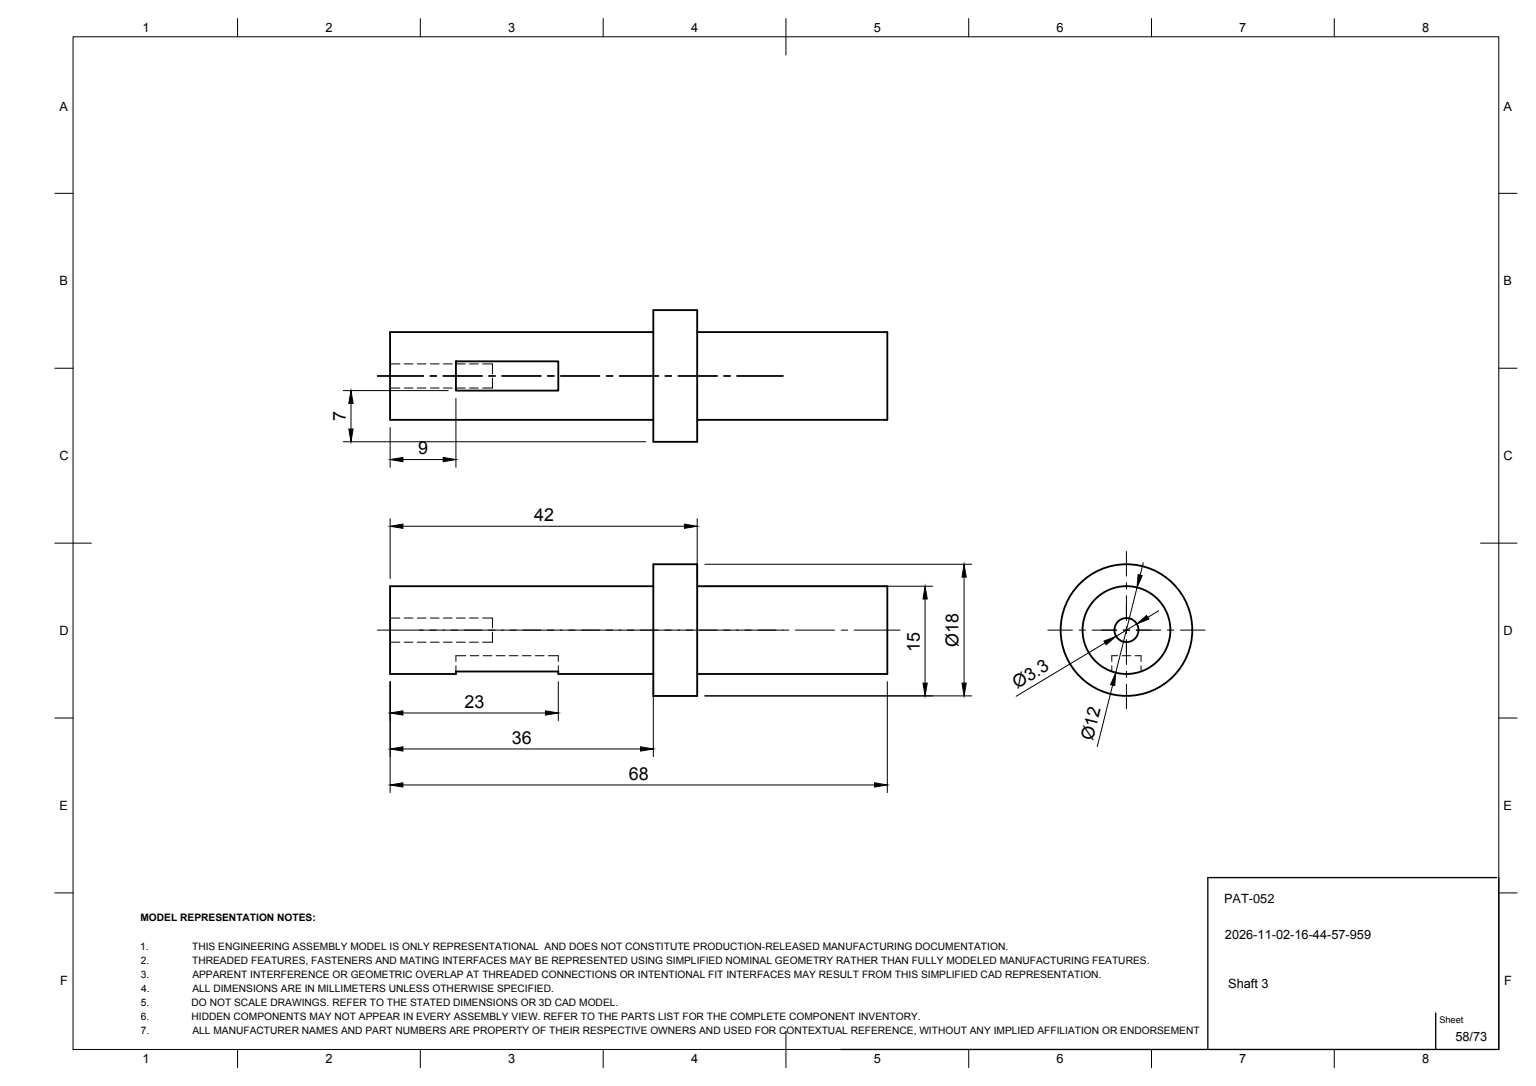
ISO-10303-21;
HEADER;
/* Generated by software containing ST-Developer
 * from STEP Tools, Inc. (www.steptools.com) 
 */

FILE_DESCRIPTION(
/* description */ ('Hand-crank gear train demonstrator'),
/* implementation_level */ '2;1');

FILE_NAME(
/* name */ 'Shaft 3.step',
/* time_stamp */ '2026-10-28T03:22:13-07:00',
/* author */ (''),
/* organization */ (''),
/* preprocessor_version */ 'ST-DEVELOPER v20.2',
/* originating_system */ 'Autodesk Translation Framework v15.17.0.0',
/* authorisation */ '');

FILE_SCHEMA (('AUTOMOTIVE_DESIGN { 1 0 10303 214 3 1 1 }'));
ENDSEC;

DATA;
#10=MECHANICAL_DESIGN_GEOMETRIC_PRESENTATION_REPRESENTATION('',(#1248),#62758);
#1105=SHAPE_REPRESENTATION_RELATIONSHIP('SRR','None',#63082,#1169);
#1169=ADVANCED_BREP_SHAPE_REPRESENTATION('',(#1323),#62736);
#1248=STYLED_ITEM('',(#63462),#1323);
#1323=MANIFOLD_SOLID_BREP('Body1',#16432);
#1586=FACE_BOUND('',#3853,.T.);
#1587=FACE_BOUND('',#3855,.T.);
#1588=FACE_BOUND('',#3859,.T.);
#1589=FACE_BOUND('',#3861,.T.);
#1957=PLANE('',#18208);
#1958=PLANE('',#18209);
#1959=PLANE('',#18210);
#1960=PLANE('',#18212);
#1961=PLANE('',#18213);
#1962=PLANE('',#18214);
#1963=PLANE('',#18216);
#1964=PLANE('',#18219);
#1965=PLANE('',#18227);
#1966=PLANE('',#18228);
#2665=FACE_OUTER_BOUND('',#3845,.T.);
#2666=FACE_OUTER_BOUND('',#3846,.T.);
#2667=FACE_OUTER_BOUND('',#3847,.T.);
#2668=FACE_OUTER_BOUND('',#3848,.T.);
#2669=FACE_OUTER_BOUND('',#3849,.T.);
#2670=FACE_OUTER_BOUND('',#3850,.T.);
#2671=FACE_OUTER_BOUND('',#3851,.T.);
#2672=FACE_OUTER_BOUND('',#3852,.T.);
#2673=FACE_OUTER_BOUND('',#3854,.T.);
#2674=FACE_OUTER_BOUND('',#3856,.T.);
#2675=FACE_OUTER_BOUND('',#3857,.T.);
#2676=FACE_OUTER_BOUND('',#3858,.T.);
#2677=FACE_OUTER_BOUND('',#3860,.T.);
#2678=FACE_OUTER_BOUND('',#3862,.T.);
#3845=EDGE_LOOP('',(#13139,#13140,#13141,#13142));
#3846=EDGE_LOOP('',(#13143));
#3847=EDGE_LOOP('',(#13144,#13145,#13146,#13147));
#3848=EDGE_LOOP('',(#13148,#13149,#13150,#13151));
#3849=EDGE_LOOP('',(#13152,#13153,#13154,#13155));
#3850=EDGE_LOOP('',(#13156,#13157,#13158,#13159));
#3851=EDGE_LOOP('',(#13160,#13161,#13162,#13163));
#3852=EDGE_LOOP('',(#13164));
#3853=EDGE_LOOP('',(#13165));
#3854=EDGE_LOOP('',(#13166));
#3855=EDGE_LOOP('',(#13167));
#3856=EDGE_LOOP('',(#13168,#13169,#13170,#13171));
#3857=EDGE_LOOP('',(#13172,#13173,#13174,#13175));
#3858=EDGE_LOOP('',(#13176,#13177,#13178,#13179));
#3859=EDGE_LOOP('',(#13180,#13181,#13182,#13183));
#3860=EDGE_LOOP('',(#13184));
#3861=EDGE_LOOP('',(#13185));
#3862=EDGE_LOOP('',(#13186));
#4955=LINE('',#26595,#6087);
#4956=LINE('',#26601,#6088);
#4957=LINE('',#26603,#6089);
#4958=LINE('',#26605,#6090);
#4959=LINE('',#26606,#6091);
#4960=LINE('',#26611,#6092);
#4961=LINE('',#26612,#6093);
#4962=LINE('',#26615,#6094);
#4963=LINE('',#26617,#6095);
#4964=LINE('',#26618,#6096);
#4965=LINE('',#26620,#6097);
#4966=LINE('',#26634,#6098);
#4967=LINE('',#26637,#6099);
#4968=LINE('',#26642,#6100);
#6087=VECTOR('',#21598,0.164999999999999);
#6088=VECTOR('',#21605,1.);
#6089=VECTOR('',#21606,1.);
#6090=VECTOR('',#21607,1.);
#6091=VECTOR('',#21608,1.);
#6092=VECTOR('',#21613,1.);
#6093=VECTOR('',#21614,1.);
#6094=VECTOR('',#21617,1.);
#6095=VECTOR('',#21618,1.);
#6096=VECTOR('',#21619,1.);
#6097=VECTOR('',#21622,1.);
#6098=VECTOR('',#21641,0.9);
#6099=VECTOR('',#21644,0.6);
#6100=VECTOR('',#21651,0.6);
#6993=CIRCLE('',#18206,0.164999999999999);
#6994=CIRCLE('',#18207,0.164999999999999);
#6995=CIRCLE('',#18211,0.6);
#6996=CIRCLE('',#18215,0.6);
#6997=CIRCLE('',#18217,0.9);
#6998=CIRCLE('',#18218,0.6);
#6999=CIRCLE('',#18220,0.9);
#7000=CIRCLE('',#18221,0.6);
#7001=CIRCLE('',#18224,0.6);
#7002=CIRCLE('',#18226,0.6);
#7994=VERTEX_POINT('',#26592);
#7995=VERTEX_POINT('',#26594);
#7996=VERTEX_POINT('',#26599);
#7997=VERTEX_POINT('',#26600);
#7998=VERTEX_POINT('',#26602);
#7999=VERTEX_POINT('',#26604);
#8000=VERTEX_POINT('',#26608);
#8001=VERTEX_POINT('',#26610);
#8002=VERTEX_POINT('',#26614);
#8003=VERTEX_POINT('',#26616);
#8004=VERTEX_POINT('',#26624);
#8005=VERTEX_POINT('',#26626);
#8006=VERTEX_POINT('',#26629);
#8007=VERTEX_POINT('',#26631);
#8008=VERTEX_POINT('',#26636);
#8009=VERTEX_POINT('',#26640);
#9821=EDGE_CURVE('',#7994,#7994,#6993,.T.);
#9822=EDGE_CURVE('',#7994,#7995,#4955,.T.);
#9823=EDGE_CURVE('',#7995,#7995,#6994,.T.);
#9824=EDGE_CURVE('',#7996,#7997,#4956,.T.);
#9825=EDGE_CURVE('',#7996,#7998,#4957,.T.);
#9826=EDGE_CURVE('',#7999,#7998,#4958,.T.);
#9827=EDGE_CURVE('',#7999,#7997,#4959,.T.);
#9828=EDGE_CURVE('',#7997,#8000,#6995,.T.);
#9829=EDGE_CURVE('',#8001,#7999,#4960,.T.);
#9830=EDGE_CURVE('',#8000,#8001,#4961,.T.);
#9831=EDGE_CURVE('',#8000,#8002,#4962,.T.);
#9832=EDGE_CURVE('',#8001,#8003,#4963,.T.);
#9833=EDGE_CURVE('',#8003,#8002,#4964,.T.);
#9834=EDGE_CURVE('',#7998,#8003,#4965,.T.);
#9835=EDGE_CURVE('',#8002,#7996,#6996,.T.);
#9836=EDGE_CURVE('',#8004,#8004,#6997,.T.);
#9837=EDGE_CURVE('',#8005,#8005,#6998,.T.);
#9838=EDGE_CURVE('',#8006,#8006,#6999,.T.);
#9839=EDGE_CURVE('',#8007,#8007,#7000,.T.);
#9840=EDGE_CURVE('',#8004,#8006,#4966,.T.);
#9841=EDGE_CURVE('',#8007,#8008,#4967,.T.);
#9842=EDGE_CURVE('',#8008,#8008,#7001,.T.);
#9843=EDGE_CURVE('',#8009,#8009,#7002,.T.);
#9844=EDGE_CURVE('',#8009,#8005,#4968,.T.);
#13139=ORIENTED_EDGE('',*,*,#9821,.F.);
#13140=ORIENTED_EDGE('',*,*,#9822,.T.);
#13141=ORIENTED_EDGE('',*,*,#9823,.F.);
#13142=ORIENTED_EDGE('',*,*,#9822,.F.);
#13143=ORIENTED_EDGE('',*,*,#9821,.T.);
#13144=ORIENTED_EDGE('',*,*,#9824,.F.);
#13145=ORIENTED_EDGE('',*,*,#9825,.T.);
#13146=ORIENTED_EDGE('',*,*,#9826,.F.);
#13147=ORIENTED_EDGE('',*,*,#9827,.T.);
#13148=ORIENTED_EDGE('',*,*,#9828,.F.);
#13149=ORIENTED_EDGE('',*,*,#9827,.F.);
#13150=ORIENTED_EDGE('',*,*,#9829,.F.);
#13151=ORIENTED_EDGE('',*,*,#9830,.F.);
#13152=ORIENTED_EDGE('',*,*,#9831,.F.);
#13153=ORIENTED_EDGE('',*,*,#9830,.T.);
#13154=ORIENTED_EDGE('',*,*,#9832,.T.);
#13155=ORIENTED_EDGE('',*,*,#9833,.T.);
#13156=ORIENTED_EDGE('',*,*,#9829,.T.);
#13157=ORIENTED_EDGE('',*,*,#9826,.T.);
#13158=ORIENTED_EDGE('',*,*,#9834,.T.);
#13159=ORIENTED_EDGE('',*,*,#9832,.F.);
#13160=ORIENTED_EDGE('',*,*,#9835,.F.);
#13161=ORIENTED_EDGE('',*,*,#9833,.F.);
#13162=ORIENTED_EDGE('',*,*,#9834,.F.);
#13163=ORIENTED_EDGE('',*,*,#9825,.F.);
#13164=ORIENTED_EDGE('',*,*,#9836,.T.);
#13165=ORIENTED_EDGE('',*,*,#9837,.F.);
#13166=ORIENTED_EDGE('',*,*,#9838,.F.);
#13167=ORIENTED_EDGE('',*,*,#9839,.F.);
#13168=ORIENTED_EDGE('',*,*,#9836,.F.);
#13169=ORIENTED_EDGE('',*,*,#9840,.T.);
#13170=ORIENTED_EDGE('',*,*,#9838,.T.);
#13171=ORIENTED_EDGE('',*,*,#9840,.F.);
#13172=ORIENTED_EDGE('',*,*,#9839,.T.);
#13173=ORIENTED_EDGE('',*,*,#9841,.T.);
#13174=ORIENTED_EDGE('',*,*,#9842,.T.);
#13175=ORIENTED_EDGE('',*,*,#9841,.F.);
#13176=ORIENTED_EDGE('',*,*,#9843,.F.);
#13177=ORIENTED_EDGE('',*,*,#9844,.T.);
#13178=ORIENTED_EDGE('',*,*,#9837,.T.);
#13179=ORIENTED_EDGE('',*,*,#9844,.F.);
#13180=ORIENTED_EDGE('',*,*,#9831,.T.);
#13181=ORIENTED_EDGE('',*,*,#9835,.T.);
#13182=ORIENTED_EDGE('',*,*,#9824,.T.);
#13183=ORIENTED_EDGE('',*,*,#9828,.T.);
#13184=ORIENTED_EDGE('',*,*,#9843,.T.);
#13185=ORIENTED_EDGE('',*,*,#9823,.T.);
#13186=ORIENTED_EDGE('',*,*,#9842,.F.);
#15331=CYLINDRICAL_SURFACE('',#18205,0.164999999999999);
#15332=CYLINDRICAL_SURFACE('',#18222,0.9);
#15333=CYLINDRICAL_SURFACE('',#18223,0.6);
#15334=CYLINDRICAL_SURFACE('',#18225,0.6);
#15975=ADVANCED_FACE('',(#2665),#15331,.F.);
#15976=ADVANCED_FACE('',(#2666),#1957,.T.);
#15977=ADVANCED_FACE('',(#2667),#1958,.F.);
#15978=ADVANCED_FACE('',(#2668),#1959,.T.);
#15979=ADVANCED_FACE('',(#2669),#1960,.F.);
#15980=ADVANCED_FACE('',(#2670),#1961,.F.);
#15981=ADVANCED_FACE('',(#2671),#1962,.F.);
#15982=ADVANCED_FACE('',(#2672,#1586),#1963,.T.);
#15983=ADVANCED_FACE('',(#2673,#1587),#1964,.F.);
#15984=ADVANCED_FACE('',(#2674),#15332,.T.);
#15985=ADVANCED_FACE('',(#2675),#15333,.T.);
#15986=ADVANCED_FACE('',(#2676,#1588),#15334,.T.);
#15987=ADVANCED_FACE('',(#2677,#1589),#1965,.T.);
#15988=ADVANCED_FACE('',(#2678),#1966,.F.);
#16432=CLOSED_SHELL('',(#15975,#15976,#15977,#15978,#15979,#15980,#15981,
#15982,#15983,#15984,#15985,#15986,#15987,#15988));
#18204=AXIS2_PLACEMENT_3D('',#26590,#21592,#21593);
#18205=AXIS2_PLACEMENT_3D('',#26591,#21594,#21595);
#18206=AXIS2_PLACEMENT_3D('',#26593,#21596,#21597);
#18207=AXIS2_PLACEMENT_3D('',#26596,#21599,#21600);
#18208=AXIS2_PLACEMENT_3D('',#26597,#21601,#21602);
#18209=AXIS2_PLACEMENT_3D('',#26598,#21603,#21604);
#18210=AXIS2_PLACEMENT_3D('',#26607,#21609,#21610);
#18211=AXIS2_PLACEMENT_3D('',#26609,#21611,#21612);
#18212=AXIS2_PLACEMENT_3D('',#26613,#21615,#21616);
#18213=AXIS2_PLACEMENT_3D('',#26619,#21620,#21621);
#18214=AXIS2_PLACEMENT_3D('',#26621,#21623,#21624);
#18215=AXIS2_PLACEMENT_3D('',#26622,#21625,#21626);
#18216=AXIS2_PLACEMENT_3D('',#26623,#21627,#21628);
#18217=AXIS2_PLACEMENT_3D('',#26625,#21629,#21630);
#18218=AXIS2_PLACEMENT_3D('',#26627,#21631,#21632);
#18219=AXIS2_PLACEMENT_3D('',#26628,#21633,#21634);
#18220=AXIS2_PLACEMENT_3D('',#26630,#21635,#21636);
#18221=AXIS2_PLACEMENT_3D('',#26632,#21637,#21638);
#18222=AXIS2_PLACEMENT_3D('',#26633,#21639,#21640);
#18223=AXIS2_PLACEMENT_3D('',#26635,#21642,#21643);
#18224=AXIS2_PLACEMENT_3D('',#26638,#21645,#21646);
#18225=AXIS2_PLACEMENT_3D('',#26639,#21647,#21648);
#18226=AXIS2_PLACEMENT_3D('',#26641,#21649,#21650);
#18227=AXIS2_PLACEMENT_3D('',#26643,#21652,#21653);
#18228=AXIS2_PLACEMENT_3D('',#26644,#21654,#21655);
#21592=DIRECTION('axis',(0.,0.,1.));
#21593=DIRECTION('refdir',(1.,0.,0.));
#21594=DIRECTION('center_axis',(0.,1.,0.));
#21595=DIRECTION('ref_axis',(1.,0.,0.));
#21596=DIRECTION('center_axis',(0.,1.,0.));
#21597=DIRECTION('ref_axis',(1.,0.,0.));
#21598=DIRECTION('',(0.,1.,0.));
#21599=DIRECTION('center_axis',(0.,-1.,0.));
#21600=DIRECTION('ref_axis',(1.,0.,0.));
#21601=DIRECTION('center_axis',(0.,1.,0.));
#21602=DIRECTION('ref_axis',(1.,0.,0.));
#21603=DIRECTION('center_axis',(-1.,0.,0.));
#21604=DIRECTION('ref_axis',(0.,0.,1.));
#21605=DIRECTION('',(0.,-1.,0.));
#21606=DIRECTION('',(0.,0.,1.));
#21607=DIRECTION('',(0.,1.,0.));
#21608=DIRECTION('',(0.,0.,-1.));
#21609=DIRECTION('center_axis',(0.,1.,0.));
#21610=DIRECTION('ref_axis',(1.,0.,0.));
#21611=DIRECTION('center_axis',(0.,-1.,0.));
#21612=DIRECTION('ref_axis',(1.,0.,0.));
#21613=DIRECTION('',(-1.,0.,0.));
#21614=DIRECTION('',(0.,0.,1.));
#21615=DIRECTION('center_axis',(1.,0.,0.));
#21616=DIRECTION('ref_axis',(0.,0.,-1.));
#21617=DIRECTION('',(0.,1.,0.));
#21618=DIRECTION('',(0.,1.,0.));
#21619=DIRECTION('',(0.,0.,-1.));
#21620=DIRECTION('center_axis',(0.,0.,1.));
#21621=DIRECTION('ref_axis',(1.,0.,0.));
#21622=DIRECTION('',(1.,0.,0.));
#21623=DIRECTION('center_axis',(0.,1.,0.));
#21624=DIRECTION('ref_axis',(0.,0.,1.));
#21625=DIRECTION('center_axis',(0.,1.,0.));
#21626=DIRECTION('ref_axis',(1.,0.,0.));
#21627=DIRECTION('center_axis',(0.,1.,0.));
#21628=DIRECTION('ref_axis',(1.,0.,0.));
#21629=DIRECTION('center_axis',(0.,1.,0.));
#21630=DIRECTION('ref_axis',(1.,0.,0.));
#21631=DIRECTION('center_axis',(0.,1.,0.));
#21632=DIRECTION('ref_axis',(1.,0.,0.));
#21633=DIRECTION('center_axis',(0.,1.,0.));
#21634=DIRECTION('ref_axis',(1.,0.,0.));
#21635=DIRECTION('center_axis',(0.,1.,0.));
#21636=DIRECTION('ref_axis',(1.,0.,0.));
#21637=DIRECTION('center_axis',(0.,-1.,0.));
#21638=DIRECTION('ref_axis',(1.,0.,0.));
#21639=DIRECTION('center_axis',(0.,1.,0.));
#21640=DIRECTION('ref_axis',(1.,0.,0.));
#21641=DIRECTION('',(0.,-1.,0.));
#21642=DIRECTION('center_axis',(0.,1.,0.));
#21643=DIRECTION('ref_axis',(1.,0.,0.));
#21644=DIRECTION('',(0.,-1.,0.));
#21645=DIRECTION('center_axis',(0.,1.,0.));
#21646=DIRECTION('ref_axis',(1.,0.,0.));
#21647=DIRECTION('center_axis',(0.,1.,0.));
#21648=DIRECTION('ref_axis',(1.,0.,0.));
#21649=DIRECTION('center_axis',(0.,1.,0.));
#21650=DIRECTION('ref_axis',(1.,0.,0.));
#21651=DIRECTION('',(0.,-1.,0.));
#21652=DIRECTION('center_axis',(0.,1.,0.));
#21653=DIRECTION('ref_axis',(1.,0.,0.));
#21654=DIRECTION('center_axis',(0.,1.,0.));
#21655=DIRECTION('ref_axis',(1.,0.,0.));
#26590=CARTESIAN_POINT('',(0.,0.,0.));
#26591=CARTESIAN_POINT('Origin',(12.,1.8,9.));
#26592=CARTESIAN_POINT('',(11.835,1.8,9.));
#26593=CARTESIAN_POINT('Origin',(12.,1.8,9.));
#26594=CARTESIAN_POINT('',(11.835,3.2,9.));
#26595=CARTESIAN_POINT('',(11.835,1.8,9.));
#26596=CARTESIAN_POINT('Origin',(12.,3.2,9.));
#26597=CARTESIAN_POINT('Origin',(12.,1.8,9.));
#26598=CARTESIAN_POINT('Origin',(11.8,0.9,7.8));
#26599=CARTESIAN_POINT('',(11.8,2.3,8.43431457505076));
#26600=CARTESIAN_POINT('',(11.8,0.9,8.43431457505076));
#26601=CARTESIAN_POINT('',(11.8,-3.6,8.43431457505076));
#26602=CARTESIAN_POINT('',(11.8,2.3,8.65));
#26603=CARTESIAN_POINT('',(11.8,2.3,8.65));
#26604=CARTESIAN_POINT('',(11.8,0.9,8.65));
#26605=CARTESIAN_POINT('',(11.8,0.9,8.65));
#26606=CARTESIAN_POINT('',(11.8,0.9,8.65));
#26607=CARTESIAN_POINT('Origin',(12.,0.9,8.225));
#26608=CARTESIAN_POINT('',(12.2,0.9,8.43431457505076));
#26609=CARTESIAN_POINT('Origin',(12.,0.9,9.));
#26610=CARTESIAN_POINT('',(12.2,0.9,8.65));
#26611=CARTESIAN_POINT('',(12.2,0.9,8.65));
#26612=CARTESIAN_POINT('',(12.2,0.9,7.8));
#26613=CARTESIAN_POINT('Origin',(12.2,0.9,8.65));
#26614=CARTESIAN_POINT('',(12.2,2.3,8.43431457505076));
#26615=CARTESIAN_POINT('',(12.2,-3.6,8.43431457505076));
#26616=CARTESIAN_POINT('',(12.2,2.3,8.65));
#26617=CARTESIAN_POINT('',(12.2,0.9,8.65));
#26618=CARTESIAN_POINT('',(12.2,2.3,7.8));
#26619=CARTESIAN_POINT('Origin',(11.8,0.9,8.65));
#26620=CARTESIAN_POINT('',(12.2,2.3,8.65));
#26621=CARTESIAN_POINT('Origin',(12.,2.3,8.225));
#26622=CARTESIAN_POINT('Origin',(12.,2.3,9.));
#26623=CARTESIAN_POINT('Origin',(12.,-0.4,9.));
#26624=CARTESIAN_POINT('',(11.1,-0.4,9.));
#26625=CARTESIAN_POINT('Origin',(12.,-0.4,9.));
#26626=CARTESIAN_POINT('',(11.4,-0.4,9.));
#26627=CARTESIAN_POINT('Origin',(12.,-0.4,9.));
#26628=CARTESIAN_POINT('Origin',(12.,-1.,9.));
#26629=CARTESIAN_POINT('',(11.1,-1.,9.));
#26630=CARTESIAN_POINT('Origin',(12.,-1.,9.));
#26631=CARTESIAN_POINT('',(11.4,-1.,9.));
#26632=CARTESIAN_POINT('Origin',(12.,-1.,9.));
#26633=CARTESIAN_POINT('Origin',(12.,-1.,9.));
#26634=CARTESIAN_POINT('',(11.1,-1.,9.));
#26635=CARTESIAN_POINT('Origin',(12.,-3.6,9.));
#26636=CARTESIAN_POINT('',(11.4,-3.6,9.));
#26637=CARTESIAN_POINT('',(11.4,-3.6,9.));
#26638=CARTESIAN_POINT('Origin',(12.,-3.6,9.));
#26639=CARTESIAN_POINT('Origin',(12.,-3.6,9.));
#26640=CARTESIAN_POINT('',(11.4,3.2,9.));
#26641=CARTESIAN_POINT('Origin',(12.,3.2,9.));
#26642=CARTESIAN_POINT('',(11.4,-3.6,9.));
#26643=CARTESIAN_POINT('Origin',(12.,3.2,9.));
#26644=CARTESIAN_POINT('Origin',(12.,-3.6,9.));
#62662=UNCERTAINTY_MEASURE_WITH_UNIT(LENGTH_MEASURE(0.001),#62759,
'DISTANCE_ACCURACY_VALUE',
'Maximum model space distance between geometric entities at asserted c
onnectivities');
#62684=UNCERTAINTY_MEASURE_WITH_UNIT(LENGTH_MEASURE(0.001),#62759,
'DISTANCE_ACCURACY_VALUE',
'Maximum model space distance between geometric entities at asserted c
onnectivities');
#62736=(
GEOMETRIC_REPRESENTATION_CONTEXT(3)
GLOBAL_UNCERTAINTY_ASSIGNED_CONTEXT((#62662))
GLOBAL_UNIT_ASSIGNED_CONTEXT((#62759,#62761,#62762))
REPRESENTATION_CONTEXT('','3D')
);
#62758=(
GEOMETRIC_REPRESENTATION_CONTEXT(3)
GLOBAL_UNCERTAINTY_ASSIGNED_CONTEXT((#62684))
GLOBAL_UNIT_ASSIGNED_CONTEXT((#62759,#62761,#62762))
REPRESENTATION_CONTEXT('','3D')
);
#62759=(
LENGTH_UNIT()
NAMED_UNIT(*)
SI_UNIT(.CENTI.,.METRE.)
);
#62761=(
NAMED_UNIT(*)
PLANE_ANGLE_UNIT()
SI_UNIT($,.RADIAN.)
);
#62762=(
NAMED_UNIT(*)
SI_UNIT($,.STERADIAN.)
SOLID_ANGLE_UNIT()
);
#62814=SHAPE_DEFINITION_REPRESENTATION(#62897,#63082);
#62897=PRODUCT_DEFINITION_SHAPE('',$,#63156);
#63082=SHAPE_REPRESENTATION('',(#18204),#62736);
#63104=PRODUCT_DEFINITION_CONTEXT('part definition',#63325,'design');
#63156=PRODUCT_DEFINITION('Shaft 3','Shaft 3',#63229,#63104);
#63229=PRODUCT_DEFINITION_FORMATION('',$,#63378);
#63325=APPLICATION_CONTEXT(
'Core Data for Automotive Mechanical Design Process');
#63326=PRODUCT_CONTEXT('part definition',#63325,'mechanical');
#63378=PRODUCT('Shaft 3','Shaft 3','Shaft 3',(#63326));
#63456=COLOUR_RGB('Grey',0.48,0.52,0.57);
#63457=FILL_AREA_STYLE_COLOUR('',#63456);
#63458=FILL_AREA_STYLE('',(#63457));
#63459=SURFACE_STYLE_FILL_AREA(#63458);
#63460=SURFACE_SIDE_STYLE('',(#63459));
#63461=SURFACE_STYLE_USAGE(.BOTH.,#63460);
#63462=PRESENTATION_STYLE_ASSIGNMENT((#63461));
ENDSEC;
END-ISO-10303-21;
